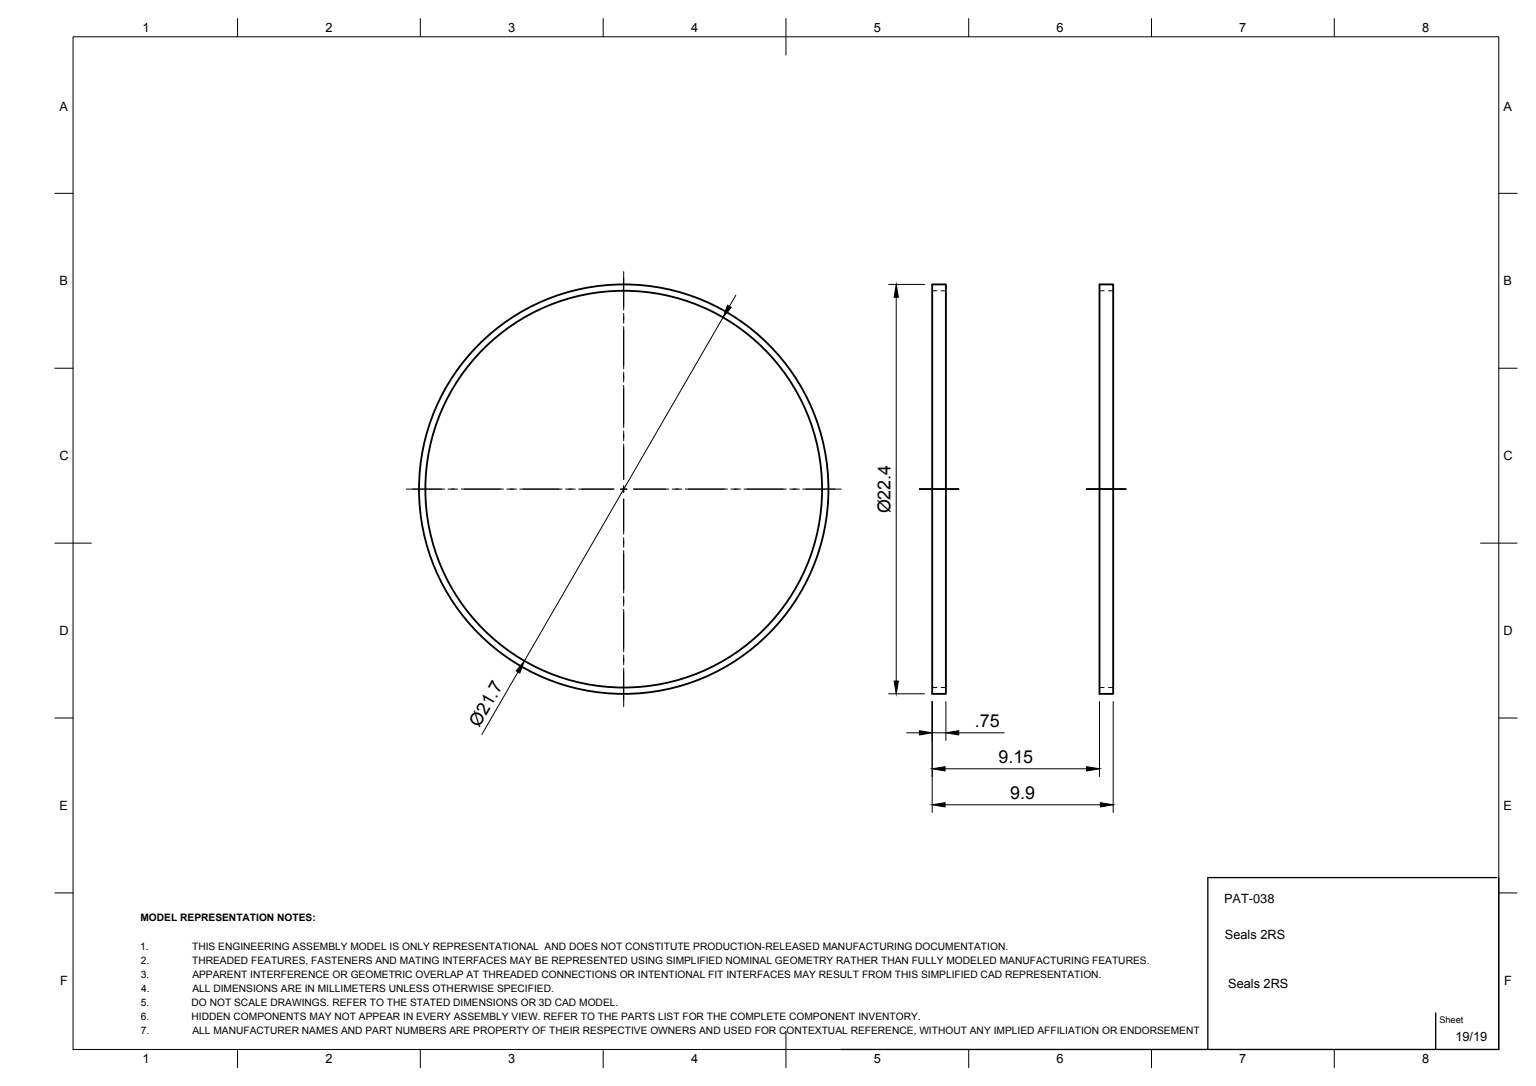
ISO-10303-21;
HEADER;
/* Generated by software containing ST-Developer
 * from STEP Tools, Inc. (www.steptools.com) 
 */

FILE_DESCRIPTION(
/* description */ ('Fork-mounted skate wheel'),
/* implementation_level */ '2;1');

FILE_NAME(
/* name */ 'Seals 2RS.step',
/* time_stamp */ '2026-10-29T16:11:26-07:00',
/* author */ (''),
/* organization */ (''),
/* preprocessor_version */ 'ST-DEVELOPER v20.2',
/* originating_system */ 'Autodesk Translation Framework v15.17.0.0',
/* authorisation */ '');

FILE_SCHEMA (('AUTOMOTIVE_DESIGN { 1 0 10303 214 3 1 1 }'));
ENDSEC;

DATA;
#10=MECHANICAL_DESIGN_GEOMETRIC_PRESENTATION_REPRESENTATION('',(#162,#163),#3688);
#132=SHAPE_REPRESENTATION_RELATIONSHIP('SRR','None',#3757,#144);
#144=ADVANCED_BREP_SHAPE_REPRESENTATION('',(#180,#181),#3686);
#162=STYLED_ITEM('',(#3896),#180);
#163=STYLED_ITEM('',(#3896),#181);
#180=MANIFOLD_SOLID_BREP('Body1',#1824);
#181=MANIFOLD_SOLID_BREP('Body2',#1825);
#213=FACE_BOUND('',#521,.T.);
#214=FACE_BOUND('',#524,.T.);
#215=FACE_BOUND('',#527,.T.);
#216=FACE_BOUND('',#530,.T.);
#270=PLANE('',#2184);
#271=PLANE('',#2189);
#272=PLANE('',#2192);
#273=PLANE('',#2197);
#377=FACE_OUTER_BOUND('',#520,.T.);
#378=FACE_OUTER_BOUND('',#522,.T.);
#379=FACE_OUTER_BOUND('',#523,.T.);
#380=FACE_OUTER_BOUND('',#525,.T.);
#381=FACE_OUTER_BOUND('',#526,.T.);
#382=FACE_OUTER_BOUND('',#528,.T.);
#383=FACE_OUTER_BOUND('',#529,.T.);
#384=FACE_OUTER_BOUND('',#531,.T.);
#520=EDGE_LOOP('',(#1625));
#521=EDGE_LOOP('',(#1626));
#522=EDGE_LOOP('',(#1627,#1628,#1629,#1630));
#523=EDGE_LOOP('',(#1631));
#524=EDGE_LOOP('',(#1632));
#525=EDGE_LOOP('',(#1633,#1634,#1635,#1636));
#526=EDGE_LOOP('',(#1637));
#527=EDGE_LOOP('',(#1638));
#528=EDGE_LOOP('',(#1639,#1640,#1641,#1642));
#529=EDGE_LOOP('',(#1643));
#530=EDGE_LOOP('',(#1644));
#531=EDGE_LOOP('',(#1645,#1646,#1647,#1648));
#626=LINE('',#3608,#720);
#627=LINE('',#3613,#721);
#628=LINE('',#3622,#722);
#629=LINE('',#3627,#723);
#720=VECTOR('',#2767,1.119765);
#721=VECTOR('',#2774,1.085235);
#722=VECTOR('',#2785,1.119765);
#723=VECTOR('',#2792,1.085235);
#828=CIRCLE('',#2185,1.119765);
#829=CIRCLE('',#2186,1.085235);
#830=CIRCLE('',#2188,1.119765);
#831=CIRCLE('',#2190,1.085235);
#832=CIRCLE('',#2193,1.119765);
#833=CIRCLE('',#2194,1.085235);
#834=CIRCLE('',#2196,1.119765);
#835=CIRCLE('',#2198,1.085235);
#983=VERTEX_POINT('',#3601);
#984=VERTEX_POINT('',#3603);
#985=VERTEX_POINT('',#3606);
#986=VERTEX_POINT('',#3610);
#987=VERTEX_POINT('',#3615);
#988=VERTEX_POINT('',#3617);
#989=VERTEX_POINT('',#3620);
#990=VERTEX_POINT('',#3624);
#1199=EDGE_CURVE('',#983,#983,#828,.T.);
#1200=EDGE_CURVE('',#984,#984,#829,.T.);
#1201=EDGE_CURVE('',#985,#985,#830,.T.);
#1202=EDGE_CURVE('',#985,#983,#626,.T.);
#1203=EDGE_CURVE('',#986,#986,#831,.T.);
#1204=EDGE_CURVE('',#986,#984,#627,.T.);
#1205=EDGE_CURVE('',#987,#987,#832,.T.);
#1206=EDGE_CURVE('',#988,#988,#833,.T.);
#1207=EDGE_CURVE('',#989,#989,#834,.T.);
#1208=EDGE_CURVE('',#989,#987,#628,.T.);
#1209=EDGE_CURVE('',#990,#990,#835,.T.);
#1210=EDGE_CURVE('',#990,#988,#629,.T.);
#1625=ORIENTED_EDGE('',*,*,#1199,.F.);
#1626=ORIENTED_EDGE('',*,*,#1200,.T.);
#1627=ORIENTED_EDGE('',*,*,#1201,.F.);
#1628=ORIENTED_EDGE('',*,*,#1202,.T.);
#1629=ORIENTED_EDGE('',*,*,#1199,.T.);
#1630=ORIENTED_EDGE('',*,*,#1202,.F.);
#1631=ORIENTED_EDGE('',*,*,#1201,.T.);
#1632=ORIENTED_EDGE('',*,*,#1203,.F.);
#1633=ORIENTED_EDGE('',*,*,#1203,.T.);
#1634=ORIENTED_EDGE('',*,*,#1204,.T.);
#1635=ORIENTED_EDGE('',*,*,#1200,.F.);
#1636=ORIENTED_EDGE('',*,*,#1204,.F.);
#1637=ORIENTED_EDGE('',*,*,#1205,.F.);
#1638=ORIENTED_EDGE('',*,*,#1206,.T.);
#1639=ORIENTED_EDGE('',*,*,#1207,.F.);
#1640=ORIENTED_EDGE('',*,*,#1208,.T.);
#1641=ORIENTED_EDGE('',*,*,#1205,.T.);
#1642=ORIENTED_EDGE('',*,*,#1208,.F.);
#1643=ORIENTED_EDGE('',*,*,#1207,.T.);
#1644=ORIENTED_EDGE('',*,*,#1209,.F.);
#1645=ORIENTED_EDGE('',*,*,#1209,.T.);
#1646=ORIENTED_EDGE('',*,*,#1210,.T.);
#1647=ORIENTED_EDGE('',*,*,#1206,.F.);
#1648=ORIENTED_EDGE('',*,*,#1210,.F.);
#1688=CYLINDRICAL_SURFACE('',#2187,1.119765);
#1689=CYLINDRICAL_SURFACE('',#2191,1.085235);
#1690=CYLINDRICAL_SURFACE('',#2195,1.119765);
#1691=CYLINDRICAL_SURFACE('',#2199,1.085235);
#1795=ADVANCED_FACE('',(#377,#213),#270,.T.);
#1796=ADVANCED_FACE('',(#378),#1688,.T.);
#1797=ADVANCED_FACE('',(#379,#214),#271,.T.);
#1798=ADVANCED_FACE('',(#380),#1689,.F.);
#1799=ADVANCED_FACE('',(#381,#215),#272,.T.);
#1800=ADVANCED_FACE('',(#382),#1690,.T.);
#1801=ADVANCED_FACE('',(#383,#216),#273,.T.);
#1802=ADVANCED_FACE('',(#384),#1691,.F.);
#1824=CLOSED_SHELL('',(#1795,#1796,#1797,#1798));
#1825=CLOSED_SHELL('',(#1799,#1800,#1801,#1802));
#2183=AXIS2_PLACEMENT_3D('',#3599,#2755,#2756);
#2184=AXIS2_PLACEMENT_3D('',#3600,#2757,#2758);
#2185=AXIS2_PLACEMENT_3D('',#3602,#2759,#2760);
#2186=AXIS2_PLACEMENT_3D('',#3604,#2761,#2762);
#2187=AXIS2_PLACEMENT_3D('',#3605,#2763,#2764);
#2188=AXIS2_PLACEMENT_3D('',#3607,#2765,#2766);
#2189=AXIS2_PLACEMENT_3D('',#3609,#2768,#2769);
#2190=AXIS2_PLACEMENT_3D('',#3611,#2770,#2771);
#2191=AXIS2_PLACEMENT_3D('',#3612,#2772,#2773);
#2192=AXIS2_PLACEMENT_3D('',#3614,#2775,#2776);
#2193=AXIS2_PLACEMENT_3D('',#3616,#2777,#2778);
#2194=AXIS2_PLACEMENT_3D('',#3618,#2779,#2780);
#2195=AXIS2_PLACEMENT_3D('',#3619,#2781,#2782);
#2196=AXIS2_PLACEMENT_3D('',#3621,#2783,#2784);
#2197=AXIS2_PLACEMENT_3D('',#3623,#2786,#2787);
#2198=AXIS2_PLACEMENT_3D('',#3625,#2788,#2789);
#2199=AXIS2_PLACEMENT_3D('',#3626,#2790,#2791);
#2755=DIRECTION('axis',(0.,0.,1.));
#2756=DIRECTION('refdir',(1.,0.,0.));
#2757=DIRECTION('center_axis',(0.,1.,0.));
#2758=DIRECTION('ref_axis',(0.,0.,1.));
#2759=DIRECTION('center_axis',(0.,-1.,0.));
#2760=DIRECTION('ref_axis',(1.,0.,0.));
#2761=DIRECTION('center_axis',(0.,-1.,0.));
#2762=DIRECTION('ref_axis',(1.,0.,0.));
#2763=DIRECTION('center_axis',(0.,-1.,0.));
#2764=DIRECTION('ref_axis',(1.,0.,0.));
#2765=DIRECTION('center_axis',(0.,-1.,0.));
#2766=DIRECTION('ref_axis',(1.,0.,0.));
#2767=DIRECTION('',(0.,1.,0.));
#2768=DIRECTION('center_axis',(0.,-1.,0.));
#2769=DIRECTION('ref_axis',(0.,0.,-1.));
#2770=DIRECTION('center_axis',(0.,-1.,0.));
#2771=DIRECTION('ref_axis',(1.,0.,0.));
#2772=DIRECTION('center_axis',(0.,-1.,0.));
#2773=DIRECTION('ref_axis',(1.,0.,0.));
#2774=DIRECTION('',(0.,1.,0.));
#2775=DIRECTION('center_axis',(0.,1.,0.));
#2776=DIRECTION('ref_axis',(0.,0.,1.));
#2777=DIRECTION('center_axis',(0.,-1.,0.));
#2778=DIRECTION('ref_axis',(1.,0.,0.));
#2779=DIRECTION('center_axis',(0.,-1.,0.));
#2780=DIRECTION('ref_axis',(1.,0.,0.));
#2781=DIRECTION('center_axis',(0.,-1.,0.));
#2782=DIRECTION('ref_axis',(1.,0.,0.));
#2783=DIRECTION('center_axis',(0.,-1.,0.));
#2784=DIRECTION('ref_axis',(1.,0.,0.));
#2785=DIRECTION('',(0.,1.,0.));
#2786=DIRECTION('center_axis',(0.,-1.,0.));
#2787=DIRECTION('ref_axis',(0.,0.,-1.));
#2788=DIRECTION('center_axis',(0.,-1.,0.));
#2789=DIRECTION('ref_axis',(1.,0.,0.));
#2790=DIRECTION('center_axis',(0.,-1.,0.));
#2791=DIRECTION('ref_axis',(1.,0.,0.));
#2792=DIRECTION('',(0.,1.,0.));
#3599=CARTESIAN_POINT('',(0.,0.,0.));
#3600=CARTESIAN_POINT('Origin',(1.119765,0.495,0.));
#3601=CARTESIAN_POINT('',(-1.119765,0.495,-1.37131662304724E-16));
#3602=CARTESIAN_POINT('Origin',(0.,0.495,0.));
#3603=CARTESIAN_POINT('',(-1.085235,0.495,-1.32902956907268E-16));
#3604=CARTESIAN_POINT('Origin',(0.,0.495,0.));
#3605=CARTESIAN_POINT('Origin',(0.,0.4575,0.));
#3606=CARTESIAN_POINT('',(-1.119765,0.42,-1.37131662304724E-16));
#3607=CARTESIAN_POINT('Origin',(0.,0.42,0.));
#3608=CARTESIAN_POINT('',(-1.119765,0.4575,-1.37131662304724E-16));
#3609=CARTESIAN_POINT('Origin',(1.085235,0.42,0.));
#3610=CARTESIAN_POINT('',(-1.085235,0.42,-1.32902956907268E-16));
#3611=CARTESIAN_POINT('Origin',(0.,0.42,0.));
#3612=CARTESIAN_POINT('Origin',(0.,0.4575,0.));
#3613=CARTESIAN_POINT('',(-1.085235,0.4575,-1.32902956907268E-16));
#3614=CARTESIAN_POINT('Origin',(1.119765,-0.42,0.));
#3615=CARTESIAN_POINT('',(-1.119765,-0.42,-1.37131662304724E-16));
#3616=CARTESIAN_POINT('Origin',(0.,-0.42,0.));
#3617=CARTESIAN_POINT('',(-1.085235,-0.42,-1.32902956907268E-16));
#3618=CARTESIAN_POINT('Origin',(0.,-0.42,0.));
#3619=CARTESIAN_POINT('Origin',(0.,-0.4575,0.));
#3620=CARTESIAN_POINT('',(-1.119765,-0.495,-1.37131662304724E-16));
#3621=CARTESIAN_POINT('Origin',(0.,-0.495,0.));
#3622=CARTESIAN_POINT('',(-1.119765,-0.4575,-1.37131662304724E-16));
#3623=CARTESIAN_POINT('Origin',(1.085235,-0.495,0.));
#3624=CARTESIAN_POINT('',(-1.085235,-0.495,-1.32902956907268E-16));
#3625=CARTESIAN_POINT('Origin',(0.,-0.495,0.));
#3626=CARTESIAN_POINT('Origin',(0.,-0.4575,0.));
#3627=CARTESIAN_POINT('',(-1.085235,-0.4575,-1.32902956907268E-16));
#3669=UNCERTAINTY_MEASURE_WITH_UNIT(LENGTH_MEASURE(0.001),#3689,
'DISTANCE_ACCURACY_VALUE',
'Maximum model space distance between geometric entities at asserted c
onnectivities');
#3671=UNCERTAINTY_MEASURE_WITH_UNIT(LENGTH_MEASURE(0.001),#3689,
'DISTANCE_ACCURACY_VALUE',
'Maximum model space distance between geometric entities at asserted c
onnectivities');
#3686=(
GEOMETRIC_REPRESENTATION_CONTEXT(3)
GLOBAL_UNCERTAINTY_ASSIGNED_CONTEXT((#3669))
GLOBAL_UNIT_ASSIGNED_CONTEXT((#3689,#3691,#3692))
REPRESENTATION_CONTEXT('','3D')
);
#3688=(
GEOMETRIC_REPRESENTATION_CONTEXT(3)
GLOBAL_UNCERTAINTY_ASSIGNED_CONTEXT((#3671))
GLOBAL_UNIT_ASSIGNED_CONTEXT((#3689,#3691,#3692))
REPRESENTATION_CONTEXT('','3D')
);
#3689=(
LENGTH_UNIT()
NAMED_UNIT(*)
SI_UNIT(.CENTI.,.METRE.)
);
#3691=(
NAMED_UNIT(*)
PLANE_ANGLE_UNIT()
SI_UNIT($,.RADIAN.)
);
#3692=(
NAMED_UNIT(*)
SI_UNIT($,.STERADIAN.)
SOLID_ANGLE_UNIT()
);
#3707=SHAPE_DEFINITION_REPRESENTATION(#3729,#3757);
#3729=PRODUCT_DEFINITION_SHAPE('',$,#3774);
#3757=SHAPE_REPRESENTATION('',(#2183),#3686);
#3759=PRODUCT_DEFINITION_CONTEXT('part definition',#3809,'design');
#3774=PRODUCT_DEFINITION('Seals 2RS','Seals 2RS',#3790,#3759);
#3790=PRODUCT_DEFINITION_FORMATION('',$,#3825);
#3809=APPLICATION_CONTEXT(
'Core Data for Automotive Mechanical Design Process');
#3810=PRODUCT_CONTEXT('part definition',#3809,'mechanical');
#3825=PRODUCT('Seals 2RS','Seals 2RS','Seals 2RS',(#3810));
#3890=COLOUR_RGB('Grey',0.48,0.52,0.57);
#3891=FILL_AREA_STYLE_COLOUR('',#3890);
#3892=FILL_AREA_STYLE('',(#3891));
#3893=SURFACE_STYLE_FILL_AREA(#3892);
#3894=SURFACE_SIDE_STYLE('',(#3893));
#3895=SURFACE_STYLE_USAGE(.BOTH.,#3894);
#3896=PRESENTATION_STYLE_ASSIGNMENT((#3895));
ENDSEC;
END-ISO-10303-21;
